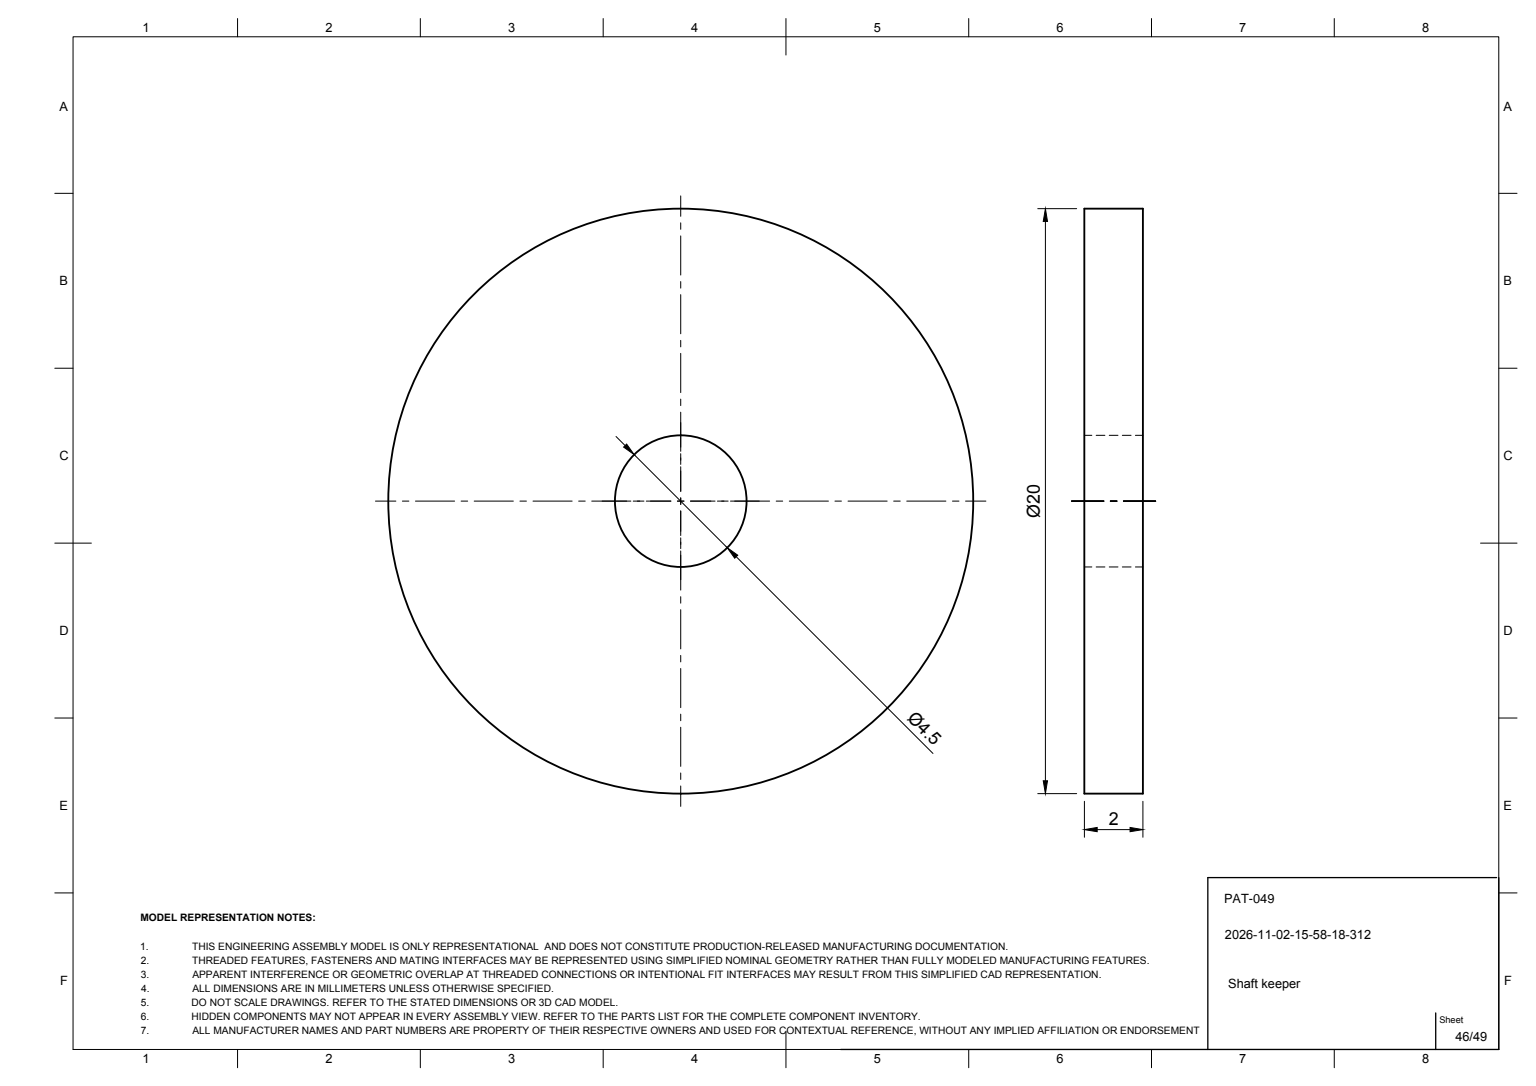
ISO-10303-21;
HEADER;
/* Generated by software containing ST-Developer
 * from STEP Tools, Inc. (www.steptools.com) 
 */

FILE_DESCRIPTION(
/* description */ ('Hand drill press frame (manual)'),
/* implementation_level */ '2;1');

FILE_NAME(
/* name */ 'Shaft keeper.step',
/* time_stamp */ '2026-10-28T03:25:28-07:00',
/* author */ (''),
/* organization */ (''),
/* preprocessor_version */ 'ST-DEVELOPER v20.2',
/* originating_system */ 'Autodesk Translation Framework v15.17.0.0',
/* authorisation */ '');

FILE_SCHEMA (('AUTOMOTIVE_DESIGN { 1 0 10303 214 3 1 1 }'));
ENDSEC;

DATA;
#10=MECHANICAL_DESIGN_GEOMETRIC_PRESENTATION_REPRESENTATION('',(#664),#33299);
#567=SHAPE_REPRESENTATION_RELATIONSHIP('SRR','None',#33529,#612);
#612=ADVANCED_BREP_SHAPE_REPRESENTATION('',(#715),#33291);
#664=STYLED_ITEM('',(#33814),#715);
#715=MANIFOLD_SOLID_BREP('Body1',#12683);
#874=FACE_BOUND('',#2736,.T.);
#875=FACE_BOUND('',#2738,.T.);
#1283=PLANE('',#14123);
#1284=PLANE('',#14124);
#1890=FACE_OUTER_BOUND('',#2733,.T.);
#1891=FACE_OUTER_BOUND('',#2734,.T.);
#1892=FACE_OUTER_BOUND('',#2735,.T.);
#1893=FACE_OUTER_BOUND('',#2737,.T.);
#2733=EDGE_LOOP('',(#11099,#11100,#11101,#11102));
#2734=EDGE_LOOP('',(#11103,#11104,#11105,#11106));
#2735=EDGE_LOOP('',(#11107));
#2736=EDGE_LOOP('',(#11108));
#2737=EDGE_LOOP('',(#11109));
#2738=EDGE_LOOP('',(#11110));
#3862=LINE('',#21337,#5027);
#3863=LINE('',#21343,#5028);
#5027=VECTOR('',#17207,0.225);
#5028=VECTOR('',#17214,1.);
#5537=CIRCLE('',#14118,0.225);
#5538=CIRCLE('',#14119,0.225);
#5539=CIRCLE('',#14121,1.);
#5540=CIRCLE('',#14122,1.);
#6513=VERTEX_POINT('',#21334);
#6514=VERTEX_POINT('',#21336);
#6515=VERTEX_POINT('',#21340);
#6516=VERTEX_POINT('',#21342);
#8078=EDGE_CURVE('',#6513,#6513,#5537,.T.);
#8079=EDGE_CURVE('',#6513,#6514,#3862,.T.);
#8080=EDGE_CURVE('',#6514,#6514,#5538,.T.);
#8081=EDGE_CURVE('',#6515,#6515,#5539,.T.);
#8082=EDGE_CURVE('',#6515,#6516,#3863,.T.);
#8083=EDGE_CURVE('',#6516,#6516,#5540,.T.);
#11099=ORIENTED_EDGE('',*,*,#8078,.F.);
#11100=ORIENTED_EDGE('',*,*,#8079,.T.);
#11101=ORIENTED_EDGE('',*,*,#8080,.T.);
#11102=ORIENTED_EDGE('',*,*,#8079,.F.);
#11103=ORIENTED_EDGE('',*,*,#8081,.F.);
#11104=ORIENTED_EDGE('',*,*,#8082,.T.);
#11105=ORIENTED_EDGE('',*,*,#8083,.T.);
#11106=ORIENTED_EDGE('',*,*,#8082,.F.);
#11107=ORIENTED_EDGE('',*,*,#8081,.T.);
#11108=ORIENTED_EDGE('',*,*,#8078,.T.);
#11109=ORIENTED_EDGE('',*,*,#8083,.F.);
#11110=ORIENTED_EDGE('',*,*,#8080,.F.);
#11914=CYLINDRICAL_SURFACE('',#14117,0.225);
#11915=CYLINDRICAL_SURFACE('',#14120,1.);
#12499=ADVANCED_FACE('',(#1890),#11914,.F.);
#12500=ADVANCED_FACE('',(#1891),#11915,.T.);
#12501=ADVANCED_FACE('',(#1892,#874),#1283,.T.);
#12502=ADVANCED_FACE('',(#1893,#875),#1284,.F.);
#12683=CLOSED_SHELL('',(#12499,#12500,#12501,#12502));
#14116=AXIS2_PLACEMENT_3D('',#21332,#17201,#17202);
#14117=AXIS2_PLACEMENT_3D('',#21333,#17203,#17204);
#14118=AXIS2_PLACEMENT_3D('',#21335,#17205,#17206);
#14119=AXIS2_PLACEMENT_3D('',#21338,#17208,#17209);
#14120=AXIS2_PLACEMENT_3D('',#21339,#17210,#17211);
#14121=AXIS2_PLACEMENT_3D('',#21341,#17212,#17213);
#14122=AXIS2_PLACEMENT_3D('',#21344,#17215,#17216);
#14123=AXIS2_PLACEMENT_3D('',#21345,#17217,#17218);
#14124=AXIS2_PLACEMENT_3D('',#21346,#17219,#17220);
#17201=DIRECTION('axis',(0.,0.,1.));
#17202=DIRECTION('refdir',(1.,0.,0.));
#17203=DIRECTION('center_axis',(0.,1.,0.));
#17204=DIRECTION('ref_axis',(1.,0.,0.));
#17205=DIRECTION('center_axis',(0.,-1.,0.));
#17206=DIRECTION('ref_axis',(1.,0.,0.));
#17207=DIRECTION('',(0.,-1.,0.));
#17208=DIRECTION('center_axis',(0.,-1.,0.));
#17209=DIRECTION('ref_axis',(1.,0.,0.));
#17210=DIRECTION('center_axis',(0.,1.,0.));
#17211=DIRECTION('ref_axis',(1.,0.,0.));
#17212=DIRECTION('center_axis',(0.,1.,0.));
#17213=DIRECTION('ref_axis',(1.,0.,0.));
#17214=DIRECTION('',(0.,-1.,0.));
#17215=DIRECTION('center_axis',(0.,1.,0.));
#17216=DIRECTION('ref_axis',(1.,0.,0.));
#17217=DIRECTION('center_axis',(0.,1.,0.));
#17218=DIRECTION('ref_axis',(1.,0.,0.));
#17219=DIRECTION('center_axis',(0.,1.,0.));
#17220=DIRECTION('ref_axis',(1.,0.,0.));
#21332=CARTESIAN_POINT('',(0.,0.,0.));
#21333=CARTESIAN_POINT('Origin',(-3.25,-5.7,20.));
#21334=CARTESIAN_POINT('',(-3.475,-5.5,20.));
#21335=CARTESIAN_POINT('Origin',(-3.25,-5.5,20.));
#21336=CARTESIAN_POINT('',(-3.475,-5.7,20.));
#21337=CARTESIAN_POINT('',(-3.475,-5.7,20.));
#21338=CARTESIAN_POINT('Origin',(-3.25,-5.7,20.));
#21339=CARTESIAN_POINT('Origin',(-3.25,-5.7,20.));
#21340=CARTESIAN_POINT('',(-4.25,-5.5,20.));
#21341=CARTESIAN_POINT('Origin',(-3.25,-5.5,20.));
#21342=CARTESIAN_POINT('',(-4.25,-5.7,20.));
#21343=CARTESIAN_POINT('',(-4.25,-5.7,20.));
#21344=CARTESIAN_POINT('Origin',(-3.25,-5.7,20.));
#21345=CARTESIAN_POINT('Origin',(-3.25,-5.5,20.));
#21346=CARTESIAN_POINT('Origin',(-3.25,-5.7,20.));
#33239=UNCERTAINTY_MEASURE_WITH_UNIT(LENGTH_MEASURE(0.001),#33300,
'DISTANCE_ACCURACY_VALUE',
'Maximum model space distance between geometric entities at asserted c
onnectivities');
#33247=UNCERTAINTY_MEASURE_WITH_UNIT(LENGTH_MEASURE(0.001),#33300,
'DISTANCE_ACCURACY_VALUE',
'Maximum model space distance between geometric entities at asserted c
onnectivities');
#33291=(
GEOMETRIC_REPRESENTATION_CONTEXT(3)
GLOBAL_UNCERTAINTY_ASSIGNED_CONTEXT((#33239))
GLOBAL_UNIT_ASSIGNED_CONTEXT((#33300,#33302,#33303))
REPRESENTATION_CONTEXT('','3D')
);
#33299=(
GEOMETRIC_REPRESENTATION_CONTEXT(3)
GLOBAL_UNCERTAINTY_ASSIGNED_CONTEXT((#33247))
GLOBAL_UNIT_ASSIGNED_CONTEXT((#33300,#33302,#33303))
REPRESENTATION_CONTEXT('','3D')
);
#33300=(
LENGTH_UNIT()
NAMED_UNIT(*)
SI_UNIT(.CENTI.,.METRE.)
);
#33302=(
NAMED_UNIT(*)
PLANE_ANGLE_UNIT()
SI_UNIT($,.RADIAN.)
);
#33303=(
NAMED_UNIT(*)
SI_UNIT($,.STERADIAN.)
SOLID_ANGLE_UNIT()
);
#33347=SHAPE_DEFINITION_REPRESENTATION(#33409,#33529);
#33409=PRODUCT_DEFINITION_SHAPE('',$,#33581);
#33529=SHAPE_REPRESENTATION('',(#14116),#33291);
#33537=PRODUCT_DEFINITION_CONTEXT('part definition',#33692,'design');
#33581=PRODUCT_DEFINITION('Shaft keeper','Shaft keeper',#33632,#33537);
#33632=PRODUCT_DEFINITION_FORMATION('',$,#33737);
#33692=APPLICATION_CONTEXT(
'Core Data for Automotive Mechanical Design Process');
#33693=PRODUCT_CONTEXT('part definition',#33692,'mechanical');
#33737=PRODUCT('Shaft keeper','Shaft keeper','Shaft keeper',(#33693));
#33808=COLOUR_RGB('Grey',0.48,0.52,0.57);
#33809=FILL_AREA_STYLE_COLOUR('',#33808);
#33810=FILL_AREA_STYLE('',(#33809));
#33811=SURFACE_STYLE_FILL_AREA(#33810);
#33812=SURFACE_SIDE_STYLE('',(#33811));
#33813=SURFACE_STYLE_USAGE(.BOTH.,#33812);
#33814=PRESENTATION_STYLE_ASSIGNMENT((#33813));
ENDSEC;
END-ISO-10303-21;
